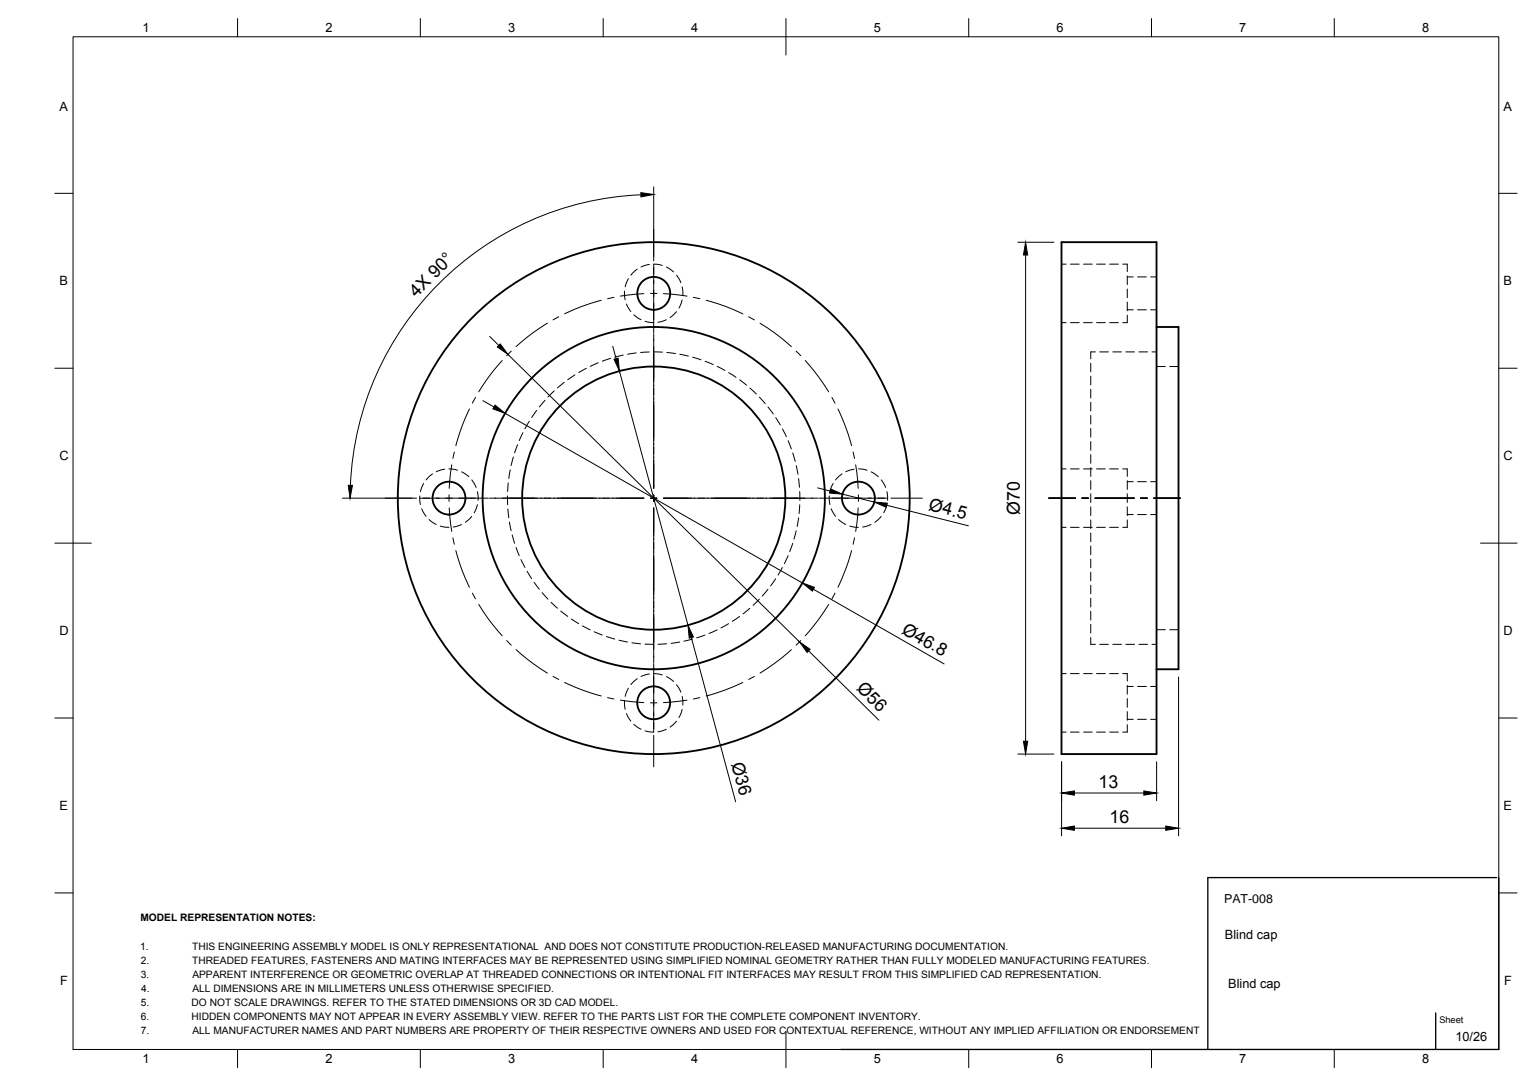
ISO-10303-21;
HEADER;
/* Generated by software containing ST-Developer
 * from STEP Tools, Inc. (www.steptools.com) 
 */

FILE_DESCRIPTION(
/* description */ ('Bearing housing with oil seal and end cap'),
/* implementation_level */ '2;1');

FILE_NAME(
/* name */ 'Blind cap.step',
/* time_stamp */ '2026-10-28T03:23:10-07:00',
/* author */ (''),
/* organization */ (''),
/* preprocessor_version */ 'ST-DEVELOPER v20.2',
/* originating_system */ 'Autodesk Translation Framework v15.17.0.0',
/* authorisation */ '');

FILE_SCHEMA (('AUTOMOTIVE_DESIGN { 1 0 10303 214 3 1 1 }'));
ENDSEC;

DATA;
#10=MECHANICAL_DESIGN_GEOMETRIC_PRESENTATION_REPRESENTATION('',(#264),#7871);
#222=SHAPE_REPRESENTATION_RELATIONSHIP('SRR','None',#7969,#243);
#243=ADVANCED_BREP_SHAPE_REPRESENTATION('',(#293),#7853);
#264=STYLED_ITEM('',(#8146),#293);
#293=MANIFOLD_SOLID_BREP('Body1',#4090);
#359=FACE_BOUND('',#921,.T.);
#360=FACE_BOUND('',#924,.T.);
#361=FACE_BOUND('',#927,.T.);
#362=FACE_BOUND('',#930,.T.);
#363=FACE_BOUND('',#936,.T.);
#364=FACE_BOUND('',#940,.T.);
#365=FACE_BOUND('',#945,.T.);
#366=FACE_BOUND('',#946,.T.);
#367=FACE_BOUND('',#947,.T.);
#368=FACE_BOUND('',#948,.T.);
#369=FACE_BOUND('',#950,.T.);
#370=FACE_BOUND('',#951,.T.);
#371=FACE_BOUND('',#952,.T.);
#372=FACE_BOUND('',#953,.T.);
#373=FACE_BOUND('',#954,.T.);
#450=PLANE('',#4499);
#451=PLANE('',#4504);
#452=PLANE('',#4509);
#453=PLANE('',#4514);
#454=PLANE('',#4524);
#455=PLANE('',#4532);
#456=PLANE('',#4535);
#457=PLANE('',#4539);
#458=PLANE('',#4540);
#624=FACE_OUTER_BOUND('',#919,.T.);
#625=FACE_OUTER_BOUND('',#920,.T.);
#626=FACE_OUTER_BOUND('',#922,.T.);
#627=FACE_OUTER_BOUND('',#923,.T.);
#628=FACE_OUTER_BOUND('',#925,.T.);
#629=FACE_OUTER_BOUND('',#926,.T.);
#630=FACE_OUTER_BOUND('',#928,.T.);
#631=FACE_OUTER_BOUND('',#929,.T.);
#632=FACE_OUTER_BOUND('',#931,.T.);
#633=FACE_OUTER_BOUND('',#932,.T.);
#634=FACE_OUTER_BOUND('',#933,.T.);
#635=FACE_OUTER_BOUND('',#934,.T.);
#636=FACE_OUTER_BOUND('',#935,.T.);
#637=FACE_OUTER_BOUND('',#937,.T.);
#638=FACE_OUTER_BOUND('',#938,.T.);
#639=FACE_OUTER_BOUND('',#939,.T.);
#640=FACE_OUTER_BOUND('',#941,.T.);
#641=FACE_OUTER_BOUND('',#942,.T.);
#642=FACE_OUTER_BOUND('',#943,.T.);
#643=FACE_OUTER_BOUND('',#944,.T.);
#644=FACE_OUTER_BOUND('',#949,.T.);
#919=EDGE_LOOP('',(#3035,#3036,#3037,#3038));
#920=EDGE_LOOP('',(#3039));
#921=EDGE_LOOP('',(#3040));
#922=EDGE_LOOP('',(#3041,#3042,#3043,#3044));
#923=EDGE_LOOP('',(#3045));
#924=EDGE_LOOP('',(#3046));
#925=EDGE_LOOP('',(#3047,#3048,#3049,#3050));
#926=EDGE_LOOP('',(#3051));
#927=EDGE_LOOP('',(#3052));
#928=EDGE_LOOP('',(#3053,#3054,#3055,#3056));
#929=EDGE_LOOP('',(#3057));
#930=EDGE_LOOP('',(#3058));
#931=EDGE_LOOP('',(#3059,#3060,#3061,#3062));
#932=EDGE_LOOP('',(#3063,#3064,#3065,#3066));
#933=EDGE_LOOP('',(#3067,#3068,#3069,#3070));
#934=EDGE_LOOP('',(#3071,#3072,#3073,#3074));
#935=EDGE_LOOP('',(#3075));
#936=EDGE_LOOP('',(#3076));
#937=EDGE_LOOP('',(#3077,#3078,#3079,#3080));
#938=EDGE_LOOP('',(#3081,#3082,#3083,#3084));
#939=EDGE_LOOP('',(#3085));
#940=EDGE_LOOP('',(#3086));
#941=EDGE_LOOP('',(#3087,#3088,#3089,#3090));
#942=EDGE_LOOP('',(#3091));
#943=EDGE_LOOP('',(#3092,#3093,#3094,#3095));
#944=EDGE_LOOP('',(#3096));
#945=EDGE_LOOP('',(#3097));
#946=EDGE_LOOP('',(#3098));
#947=EDGE_LOOP('',(#3099));
#948=EDGE_LOOP('',(#3100));
#949=EDGE_LOOP('',(#3101));
#950=EDGE_LOOP('',(#3102));
#951=EDGE_LOOP('',(#3103));
#952=EDGE_LOOP('',(#3104));
#953=EDGE_LOOP('',(#3105));
#954=EDGE_LOOP('',(#3106));
#1225=LINE('',#6532,#1487);
#1226=LINE('',#6541,#1488);
#1227=LINE('',#6550,#1489);
#1228=LINE('',#6559,#1490);
#1229=LINE('',#6567,#1491);
#1230=LINE('',#6571,#1492);
#1231=LINE('',#6575,#1493);
#1232=LINE('',#6579,#1494);
#1233=LINE('',#6587,#1495);
#1234=LINE('',#6593,#1496);
#1235=LINE('',#6598,#1497);
#1236=LINE('',#6605,#1498);
#1487=VECTOR('',#5258,0.4);
#1488=VECTOR('',#5269,0.4);
#1489=VECTOR('',#5280,0.4);
#1490=VECTOR('',#5291,0.4);
#1491=VECTOR('',#5302,0.225);
#1492=VECTOR('',#5307,0.225);
#1493=VECTOR('',#5312,0.225);
#1494=VECTOR('',#5317,0.225);
#1495=VECTOR('',#5326,1.8);
#1496=VECTOR('',#5333,2.34);
#1497=VECTOR('',#5340,2.);
#1498=VECTOR('',#5349,3.5);
#1739=CIRCLE('',#4497,0.4);
#1740=CIRCLE('',#4498,0.4);
#1741=CIRCLE('',#4500,0.225);
#1742=CIRCLE('',#4502,0.4);
#1743=CIRCLE('',#4503,0.4);
#1744=CIRCLE('',#4505,0.225);
#1745=CIRCLE('',#4507,0.4);
#1746=CIRCLE('',#4508,0.4);
#1747=CIRCLE('',#4510,0.225);
#1748=CIRCLE('',#4512,0.4);
#1749=CIRCLE('',#4513,0.4);
#1750=CIRCLE('',#4515,0.225);
#1751=CIRCLE('',#4517,0.225);
#1752=CIRCLE('',#4519,0.225);
#1753=CIRCLE('',#4521,0.225);
#1754=CIRCLE('',#4523,0.225);
#1755=CIRCLE('',#4525,2.);
#1756=CIRCLE('',#4526,1.8);
#1757=CIRCLE('',#4528,1.8);
#1758=CIRCLE('',#4530,2.34);
#1759=CIRCLE('',#4531,2.34);
#1760=CIRCLE('',#4534,2.);
#1761=CIRCLE('',#4537,3.5);
#1762=CIRCLE('',#4538,3.5);
#1987=VERTEX_POINT('',#6529);
#1988=VERTEX_POINT('',#6531);
#1989=VERTEX_POINT('',#6535);
#1990=VERTEX_POINT('',#6538);
#1991=VERTEX_POINT('',#6540);
#1992=VERTEX_POINT('',#6544);
#1993=VERTEX_POINT('',#6547);
#1994=VERTEX_POINT('',#6549);
#1995=VERTEX_POINT('',#6553);
#1996=VERTEX_POINT('',#6556);
#1997=VERTEX_POINT('',#6558);
#1998=VERTEX_POINT('',#6562);
#1999=VERTEX_POINT('',#6565);
#2000=VERTEX_POINT('',#6569);
#2001=VERTEX_POINT('',#6573);
#2002=VERTEX_POINT('',#6577);
#2003=VERTEX_POINT('',#6581);
#2004=VERTEX_POINT('',#6583);
#2005=VERTEX_POINT('',#6586);
#2006=VERTEX_POINT('',#6590);
#2007=VERTEX_POINT('',#6592);
#2008=VERTEX_POINT('',#6597);
#2009=VERTEX_POINT('',#6602);
#2010=VERTEX_POINT('',#6604);
#2381=EDGE_CURVE('',#1987,#1987,#1739,.T.);
#2382=EDGE_CURVE('',#1987,#1988,#1225,.T.);
#2383=EDGE_CURVE('',#1988,#1988,#1740,.T.);
#2384=EDGE_CURVE('',#1989,#1989,#1741,.T.);
#2385=EDGE_CURVE('',#1990,#1990,#1742,.T.);
#2386=EDGE_CURVE('',#1990,#1991,#1226,.T.);
#2387=EDGE_CURVE('',#1991,#1991,#1743,.T.);
#2388=EDGE_CURVE('',#1992,#1992,#1744,.T.);
#2389=EDGE_CURVE('',#1993,#1993,#1745,.T.);
#2390=EDGE_CURVE('',#1993,#1994,#1227,.T.);
#2391=EDGE_CURVE('',#1994,#1994,#1746,.T.);
#2392=EDGE_CURVE('',#1995,#1995,#1747,.T.);
#2393=EDGE_CURVE('',#1996,#1996,#1748,.T.);
#2394=EDGE_CURVE('',#1996,#1997,#1228,.T.);
#2395=EDGE_CURVE('',#1997,#1997,#1749,.T.);
#2396=EDGE_CURVE('',#1998,#1998,#1750,.T.);
#2397=EDGE_CURVE('',#1999,#1999,#1751,.T.);
#2398=EDGE_CURVE('',#1999,#1989,#1229,.T.);
#2399=EDGE_CURVE('',#2000,#2000,#1752,.T.);
#2400=EDGE_CURVE('',#2000,#1992,#1230,.T.);
#2401=EDGE_CURVE('',#2001,#2001,#1753,.T.);
#2402=EDGE_CURVE('',#2001,#1995,#1231,.T.);
#2403=EDGE_CURVE('',#2002,#2002,#1754,.T.);
#2404=EDGE_CURVE('',#2002,#1998,#1232,.T.);
#2405=EDGE_CURVE('',#2003,#2003,#1755,.T.);
#2406=EDGE_CURVE('',#2004,#2004,#1756,.T.);
#2407=EDGE_CURVE('',#2004,#2005,#1233,.T.);
#2408=EDGE_CURVE('',#2005,#2005,#1757,.T.);
#2409=EDGE_CURVE('',#2006,#2006,#1758,.T.);
#2410=EDGE_CURVE('',#2006,#2007,#1234,.T.);
#2411=EDGE_CURVE('',#2007,#2007,#1759,.T.);
#2412=EDGE_CURVE('',#2003,#2008,#1235,.T.);
#2413=EDGE_CURVE('',#2008,#2008,#1760,.T.);
#2414=EDGE_CURVE('',#2009,#2009,#1761,.T.);
#2415=EDGE_CURVE('',#2009,#2010,#1236,.T.);
#2416=EDGE_CURVE('',#2010,#2010,#1762,.T.);
#3035=ORIENTED_EDGE('',*,*,#2381,.F.);
#3036=ORIENTED_EDGE('',*,*,#2382,.T.);
#3037=ORIENTED_EDGE('',*,*,#2383,.F.);
#3038=ORIENTED_EDGE('',*,*,#2382,.F.);
#3039=ORIENTED_EDGE('',*,*,#2381,.T.);
#3040=ORIENTED_EDGE('',*,*,#2384,.F.);
#3041=ORIENTED_EDGE('',*,*,#2385,.F.);
#3042=ORIENTED_EDGE('',*,*,#2386,.T.);
#3043=ORIENTED_EDGE('',*,*,#2387,.F.);
#3044=ORIENTED_EDGE('',*,*,#2386,.F.);
#3045=ORIENTED_EDGE('',*,*,#2385,.T.);
#3046=ORIENTED_EDGE('',*,*,#2388,.F.);
#3047=ORIENTED_EDGE('',*,*,#2389,.F.);
#3048=ORIENTED_EDGE('',*,*,#2390,.T.);
#3049=ORIENTED_EDGE('',*,*,#2391,.F.);
#3050=ORIENTED_EDGE('',*,*,#2390,.F.);
#3051=ORIENTED_EDGE('',*,*,#2389,.T.);
#3052=ORIENTED_EDGE('',*,*,#2392,.F.);
#3053=ORIENTED_EDGE('',*,*,#2393,.F.);
#3054=ORIENTED_EDGE('',*,*,#2394,.T.);
#3055=ORIENTED_EDGE('',*,*,#2395,.F.);
#3056=ORIENTED_EDGE('',*,*,#2394,.F.);
#3057=ORIENTED_EDGE('',*,*,#2393,.T.);
#3058=ORIENTED_EDGE('',*,*,#2396,.F.);
#3059=ORIENTED_EDGE('',*,*,#2397,.F.);
#3060=ORIENTED_EDGE('',*,*,#2398,.T.);
#3061=ORIENTED_EDGE('',*,*,#2384,.T.);
#3062=ORIENTED_EDGE('',*,*,#2398,.F.);
#3063=ORIENTED_EDGE('',*,*,#2399,.F.);
#3064=ORIENTED_EDGE('',*,*,#2400,.T.);
#3065=ORIENTED_EDGE('',*,*,#2388,.T.);
#3066=ORIENTED_EDGE('',*,*,#2400,.F.);
#3067=ORIENTED_EDGE('',*,*,#2401,.F.);
#3068=ORIENTED_EDGE('',*,*,#2402,.T.);
#3069=ORIENTED_EDGE('',*,*,#2392,.T.);
#3070=ORIENTED_EDGE('',*,*,#2402,.F.);
#3071=ORIENTED_EDGE('',*,*,#2403,.F.);
#3072=ORIENTED_EDGE('',*,*,#2404,.T.);
#3073=ORIENTED_EDGE('',*,*,#2396,.T.);
#3074=ORIENTED_EDGE('',*,*,#2404,.F.);
#3075=ORIENTED_EDGE('',*,*,#2405,.T.);
#3076=ORIENTED_EDGE('',*,*,#2406,.T.);
#3077=ORIENTED_EDGE('',*,*,#2406,.F.);
#3078=ORIENTED_EDGE('',*,*,#2407,.T.);
#3079=ORIENTED_EDGE('',*,*,#2408,.T.);
#3080=ORIENTED_EDGE('',*,*,#2407,.F.);
#3081=ORIENTED_EDGE('',*,*,#2409,.F.);
#3082=ORIENTED_EDGE('',*,*,#2410,.T.);
#3083=ORIENTED_EDGE('',*,*,#2411,.T.);
#3084=ORIENTED_EDGE('',*,*,#2410,.F.);
#3085=ORIENTED_EDGE('',*,*,#2411,.F.);
#3086=ORIENTED_EDGE('',*,*,#2408,.F.);
#3087=ORIENTED_EDGE('',*,*,#2405,.F.);
#3088=ORIENTED_EDGE('',*,*,#2412,.T.);
#3089=ORIENTED_EDGE('',*,*,#2413,.T.);
#3090=ORIENTED_EDGE('',*,*,#2412,.F.);
#3091=ORIENTED_EDGE('',*,*,#2413,.F.);
#3092=ORIENTED_EDGE('',*,*,#2414,.F.);
#3093=ORIENTED_EDGE('',*,*,#2415,.T.);
#3094=ORIENTED_EDGE('',*,*,#2416,.T.);
#3095=ORIENTED_EDGE('',*,*,#2415,.F.);
#3096=ORIENTED_EDGE('',*,*,#2414,.T.);
#3097=ORIENTED_EDGE('',*,*,#2395,.T.);
#3098=ORIENTED_EDGE('',*,*,#2391,.T.);
#3099=ORIENTED_EDGE('',*,*,#2387,.T.);
#3100=ORIENTED_EDGE('',*,*,#2383,.T.);
#3101=ORIENTED_EDGE('',*,*,#2416,.F.);
#3102=ORIENTED_EDGE('',*,*,#2409,.T.);
#3103=ORIENTED_EDGE('',*,*,#2403,.T.);
#3104=ORIENTED_EDGE('',*,*,#2401,.T.);
#3105=ORIENTED_EDGE('',*,*,#2399,.T.);
#3106=ORIENTED_EDGE('',*,*,#2397,.T.);
#3789=CYLINDRICAL_SURFACE('',#4496,0.4);
#3790=CYLINDRICAL_SURFACE('',#4501,0.4);
#3791=CYLINDRICAL_SURFACE('',#4506,0.4);
#3792=CYLINDRICAL_SURFACE('',#4511,0.4);
#3793=CYLINDRICAL_SURFACE('',#4516,0.225);
#3794=CYLINDRICAL_SURFACE('',#4518,0.225);
#3795=CYLINDRICAL_SURFACE('',#4520,0.225);
#3796=CYLINDRICAL_SURFACE('',#4522,0.225);
#3797=CYLINDRICAL_SURFACE('',#4527,1.8);
#3798=CYLINDRICAL_SURFACE('',#4529,2.34);
#3799=CYLINDRICAL_SURFACE('',#4533,2.);
#3800=CYLINDRICAL_SURFACE('',#4536,3.5);
#3906=ADVANCED_FACE('',(#624),#3789,.F.);
#3907=ADVANCED_FACE('',(#625,#359),#450,.T.);
#3908=ADVANCED_FACE('',(#626),#3790,.F.);
#3909=ADVANCED_FACE('',(#627,#360),#451,.T.);
#3910=ADVANCED_FACE('',(#628),#3791,.F.);
#3911=ADVANCED_FACE('',(#629,#361),#452,.T.);
#3912=ADVANCED_FACE('',(#630),#3792,.F.);
#3913=ADVANCED_FACE('',(#631,#362),#453,.T.);
#3914=ADVANCED_FACE('',(#632),#3793,.F.);
#3915=ADVANCED_FACE('',(#633),#3794,.F.);
#3916=ADVANCED_FACE('',(#634),#3795,.F.);
#3917=ADVANCED_FACE('',(#635),#3796,.F.);
#3918=ADVANCED_FACE('',(#636,#363),#454,.T.);
#3919=ADVANCED_FACE('',(#637),#3797,.F.);
#3920=ADVANCED_FACE('',(#638),#3798,.T.);
#3921=ADVANCED_FACE('',(#639,#364),#455,.F.);
#3922=ADVANCED_FACE('',(#640),#3799,.F.);
#3923=ADVANCED_FACE('',(#641),#456,.F.);
#3924=ADVANCED_FACE('',(#642),#3800,.T.);
#3925=ADVANCED_FACE('',(#643,#365,#366,#367,#368),#457,.T.);
#3926=ADVANCED_FACE('',(#644,#369,#370,#371,#372,#373),#458,.F.);
#4090=CLOSED_SHELL('',(#3906,#3907,#3908,#3909,#3910,#3911,#3912,#3913,
#3914,#3915,#3916,#3917,#3918,#3919,#3920,#3921,#3922,#3923,#3924,#3925,
#3926));
#4495=AXIS2_PLACEMENT_3D('',#6527,#5252,#5253);
#4496=AXIS2_PLACEMENT_3D('',#6528,#5254,#5255);
#4497=AXIS2_PLACEMENT_3D('',#6530,#5256,#5257);
#4498=AXIS2_PLACEMENT_3D('',#6533,#5259,#5260);
#4499=AXIS2_PLACEMENT_3D('',#6534,#5261,#5262);
#4500=AXIS2_PLACEMENT_3D('',#6536,#5263,#5264);
#4501=AXIS2_PLACEMENT_3D('',#6537,#5265,#5266);
#4502=AXIS2_PLACEMENT_3D('',#6539,#5267,#5268);
#4503=AXIS2_PLACEMENT_3D('',#6542,#5270,#5271);
#4504=AXIS2_PLACEMENT_3D('',#6543,#5272,#5273);
#4505=AXIS2_PLACEMENT_3D('',#6545,#5274,#5275);
#4506=AXIS2_PLACEMENT_3D('',#6546,#5276,#5277);
#4507=AXIS2_PLACEMENT_3D('',#6548,#5278,#5279);
#4508=AXIS2_PLACEMENT_3D('',#6551,#5281,#5282);
#4509=AXIS2_PLACEMENT_3D('',#6552,#5283,#5284);
#4510=AXIS2_PLACEMENT_3D('',#6554,#5285,#5286);
#4511=AXIS2_PLACEMENT_3D('',#6555,#5287,#5288);
#4512=AXIS2_PLACEMENT_3D('',#6557,#5289,#5290);
#4513=AXIS2_PLACEMENT_3D('',#6560,#5292,#5293);
#4514=AXIS2_PLACEMENT_3D('',#6561,#5294,#5295);
#4515=AXIS2_PLACEMENT_3D('',#6563,#5296,#5297);
#4516=AXIS2_PLACEMENT_3D('',#6564,#5298,#5299);
#4517=AXIS2_PLACEMENT_3D('',#6566,#5300,#5301);
#4518=AXIS2_PLACEMENT_3D('',#6568,#5303,#5304);
#4519=AXIS2_PLACEMENT_3D('',#6570,#5305,#5306);
#4520=AXIS2_PLACEMENT_3D('',#6572,#5308,#5309);
#4521=AXIS2_PLACEMENT_3D('',#6574,#5310,#5311);
#4522=AXIS2_PLACEMENT_3D('',#6576,#5313,#5314);
#4523=AXIS2_PLACEMENT_3D('',#6578,#5315,#5316);
#4524=AXIS2_PLACEMENT_3D('',#6580,#5318,#5319);
#4525=AXIS2_PLACEMENT_3D('',#6582,#5320,#5321);
#4526=AXIS2_PLACEMENT_3D('',#6584,#5322,#5323);
#4527=AXIS2_PLACEMENT_3D('',#6585,#5324,#5325);
#4528=AXIS2_PLACEMENT_3D('',#6588,#5327,#5328);
#4529=AXIS2_PLACEMENT_3D('',#6589,#5329,#5330);
#4530=AXIS2_PLACEMENT_3D('',#6591,#5331,#5332);
#4531=AXIS2_PLACEMENT_3D('',#6594,#5334,#5335);
#4532=AXIS2_PLACEMENT_3D('',#6595,#5336,#5337);
#4533=AXIS2_PLACEMENT_3D('',#6596,#5338,#5339);
#4534=AXIS2_PLACEMENT_3D('',#6599,#5341,#5342);
#4535=AXIS2_PLACEMENT_3D('',#6600,#5343,#5344);
#4536=AXIS2_PLACEMENT_3D('',#6601,#5345,#5346);
#4537=AXIS2_PLACEMENT_3D('',#6603,#5347,#5348);
#4538=AXIS2_PLACEMENT_3D('',#6606,#5350,#5351);
#4539=AXIS2_PLACEMENT_3D('',#6607,#5352,#5353);
#4540=AXIS2_PLACEMENT_3D('',#6608,#5354,#5355);
#5252=DIRECTION('axis',(0.,0.,1.));
#5253=DIRECTION('refdir',(1.,0.,0.));
#5254=DIRECTION('center_axis',(0.,1.,0.));
#5255=DIRECTION('ref_axis',(1.,0.,0.));
#5256=DIRECTION('center_axis',(0.,1.,0.));
#5257=DIRECTION('ref_axis',(1.,0.,0.));
#5258=DIRECTION('',(0.,1.,0.));
#5259=DIRECTION('center_axis',(0.,-1.,0.));
#5260=DIRECTION('ref_axis',(1.,0.,0.));
#5261=DIRECTION('center_axis',(0.,1.,0.));
#5262=DIRECTION('ref_axis',(1.,0.,0.));
#5263=DIRECTION('center_axis',(0.,1.,0.));
#5264=DIRECTION('ref_axis',(1.,0.,0.));
#5265=DIRECTION('center_axis',(0.,1.,0.));
#5266=DIRECTION('ref_axis',(1.,0.,0.));
#5267=DIRECTION('center_axis',(0.,1.,0.));
#5268=DIRECTION('ref_axis',(1.,0.,0.));
#5269=DIRECTION('',(0.,1.,0.));
#5270=DIRECTION('center_axis',(0.,-1.,0.));
#5271=DIRECTION('ref_axis',(1.,0.,0.));
#5272=DIRECTION('center_axis',(0.,1.,0.));
#5273=DIRECTION('ref_axis',(1.,0.,0.));
#5274=DIRECTION('center_axis',(0.,1.,0.));
#5275=DIRECTION('ref_axis',(1.,0.,0.));
#5276=DIRECTION('center_axis',(0.,1.,0.));
#5277=DIRECTION('ref_axis',(1.,0.,0.));
#5278=DIRECTION('center_axis',(0.,1.,0.));
#5279=DIRECTION('ref_axis',(1.,0.,0.));
#5280=DIRECTION('',(0.,1.,0.));
#5281=DIRECTION('center_axis',(0.,-1.,0.));
#5282=DIRECTION('ref_axis',(1.,0.,0.));
#5283=DIRECTION('center_axis',(0.,1.,0.));
#5284=DIRECTION('ref_axis',(1.,0.,0.));
#5285=DIRECTION('center_axis',(0.,1.,0.));
#5286=DIRECTION('ref_axis',(1.,0.,0.));
#5287=DIRECTION('center_axis',(0.,1.,0.));
#5288=DIRECTION('ref_axis',(1.,0.,0.));
#5289=DIRECTION('center_axis',(0.,1.,0.));
#5290=DIRECTION('ref_axis',(1.,0.,0.));
#5291=DIRECTION('',(0.,1.,0.));
#5292=DIRECTION('center_axis',(0.,-1.,0.));
#5293=DIRECTION('ref_axis',(1.,0.,0.));
#5294=DIRECTION('center_axis',(0.,1.,0.));
#5295=DIRECTION('ref_axis',(1.,0.,0.));
#5296=DIRECTION('center_axis',(0.,1.,0.));
#5297=DIRECTION('ref_axis',(1.,0.,0.));
#5298=DIRECTION('center_axis',(0.,1.,0.));
#5299=DIRECTION('ref_axis',(1.,0.,0.));
#5300=DIRECTION('center_axis',(0.,1.,0.));
#5301=DIRECTION('ref_axis',(1.,0.,0.));
#5302=DIRECTION('',(0.,1.,0.));
#5303=DIRECTION('center_axis',(0.,1.,0.));
#5304=DIRECTION('ref_axis',(1.,0.,0.));
#5305=DIRECTION('center_axis',(0.,1.,0.));
#5306=DIRECTION('ref_axis',(1.,0.,0.));
#5307=DIRECTION('',(0.,1.,0.));
#5308=DIRECTION('center_axis',(0.,1.,0.));
#5309=DIRECTION('ref_axis',(1.,0.,0.));
#5310=DIRECTION('center_axis',(0.,1.,0.));
#5311=DIRECTION('ref_axis',(1.,0.,0.));
#5312=DIRECTION('',(0.,1.,0.));
#5313=DIRECTION('center_axis',(0.,1.,0.));
#5314=DIRECTION('ref_axis',(1.,0.,0.));
#5315=DIRECTION('center_axis',(0.,1.,0.));
#5316=DIRECTION('ref_axis',(1.,0.,0.));
#5317=DIRECTION('',(0.,1.,0.));
#5318=DIRECTION('center_axis',(0.,1.,0.));
#5319=DIRECTION('ref_axis',(1.,0.,0.));
#5320=DIRECTION('center_axis',(0.,1.,0.));
#5321=DIRECTION('ref_axis',(1.,0.,0.));
#5322=DIRECTION('center_axis',(0.,-1.,0.));
#5323=DIRECTION('ref_axis',(1.,0.,0.));
#5324=DIRECTION('center_axis',(0.,1.,0.));
#5325=DIRECTION('ref_axis',(1.,0.,0.));
#5326=DIRECTION('',(0.,-1.,0.));
#5327=DIRECTION('center_axis',(0.,-1.,0.));
#5328=DIRECTION('ref_axis',(1.,0.,0.));
#5329=DIRECTION('center_axis',(0.,1.,0.));
#5330=DIRECTION('ref_axis',(1.,0.,0.));
#5331=DIRECTION('center_axis',(0.,1.,0.));
#5332=DIRECTION('ref_axis',(1.,0.,0.));
#5333=DIRECTION('',(0.,-1.,0.));
#5334=DIRECTION('center_axis',(0.,1.,0.));
#5335=DIRECTION('ref_axis',(1.,0.,0.));
#5336=DIRECTION('center_axis',(0.,1.,0.));
#5337=DIRECTION('ref_axis',(1.,0.,0.));
#5338=DIRECTION('center_axis',(0.,1.,0.));
#5339=DIRECTION('ref_axis',(1.,0.,0.));
#5340=DIRECTION('',(0.,1.,0.));
#5341=DIRECTION('center_axis',(0.,1.,0.));
#5342=DIRECTION('ref_axis',(1.,0.,0.));
#5343=DIRECTION('center_axis',(0.,1.,0.));
#5344=DIRECTION('ref_axis',(1.,0.,0.));
#5345=DIRECTION('center_axis',(0.,1.,0.));
#5346=DIRECTION('ref_axis',(1.,0.,0.));
#5347=DIRECTION('center_axis',(0.,1.,0.));
#5348=DIRECTION('ref_axis',(1.,0.,0.));
#5349=DIRECTION('',(0.,-1.,0.));
#5350=DIRECTION('center_axis',(0.,1.,0.));
#5351=DIRECTION('ref_axis',(1.,0.,0.));
#5352=DIRECTION('center_axis',(0.,1.,0.));
#5353=DIRECTION('ref_axis',(1.,0.,0.));
#5354=DIRECTION('center_axis',(0.,1.,0.));
#5355=DIRECTION('ref_axis',(1.,0.,0.));
#6527=CARTESIAN_POINT('',(0.,0.,0.));
#6528=CARTESIAN_POINT('Origin',(-2.8,6.4,4.5));
#6529=CARTESIAN_POINT('',(-3.2,6.4,4.5));
#6530=CARTESIAN_POINT('Origin',(-2.8,6.4,4.5));
#6531=CARTESIAN_POINT('',(-3.2,7.3,4.5));
#6532=CARTESIAN_POINT('',(-3.2,6.4,4.5));
#6533=CARTESIAN_POINT('Origin',(-2.8,7.3,4.5));
#6534=CARTESIAN_POINT('Origin',(-2.8,6.4,4.5));
#6535=CARTESIAN_POINT('',(-3.025,6.4,4.5));
#6536=CARTESIAN_POINT('Origin',(-2.8,6.4,4.5));
#6537=CARTESIAN_POINT('Origin',(1.71450551880629E-16,6.4,7.3));
#6538=CARTESIAN_POINT('',(-0.4,6.4,7.3));
#6539=CARTESIAN_POINT('Origin',(1.71450551880629E-16,6.4,7.3));
#6540=CARTESIAN_POINT('',(-0.4,7.3,7.3));
#6541=CARTESIAN_POINT('',(-0.4,6.4,7.3));
#6542=CARTESIAN_POINT('Origin',(1.71450551880629E-16,7.3,7.3));
#6543=CARTESIAN_POINT('Origin',(1.66533453693773E-16,6.4,7.3));
#6544=CARTESIAN_POINT('',(-0.225,6.4,7.3));
#6545=CARTESIAN_POINT('Origin',(1.71450551880629E-16,6.4,7.3));
#6546=CARTESIAN_POINT('Origin',(2.8,6.4,4.5));
#6547=CARTESIAN_POINT('',(2.4,6.4,4.5));
#6548=CARTESIAN_POINT('Origin',(2.8,6.4,4.5));
#6549=CARTESIAN_POINT('',(2.4,7.3,4.5));
#6550=CARTESIAN_POINT('',(2.4,6.4,4.5));
#6551=CARTESIAN_POINT('Origin',(2.8,7.3,4.5));
#6552=CARTESIAN_POINT('Origin',(2.8,6.4,4.5));
#6553=CARTESIAN_POINT('',(2.575,6.4,4.5));
#6554=CARTESIAN_POINT('Origin',(2.8,6.4,4.5));
#6555=CARTESIAN_POINT('Origin',(-5.14351655641888E-16,6.4,1.7));
#6556=CARTESIAN_POINT('',(-0.400000000000001,6.4,1.7));
#6557=CARTESIAN_POINT('Origin',(-5.14351655641888E-16,6.4,1.7));
#6558=CARTESIAN_POINT('',(-0.400000000000001,7.3,1.7));
#6559=CARTESIAN_POINT('',(-0.400000000000001,6.4,1.7));
#6560=CARTESIAN_POINT('Origin',(-5.14351655641888E-16,7.3,1.7));
#6561=CARTESIAN_POINT('Origin',(-4.9960036108132E-16,6.4,1.7));
#6562=CARTESIAN_POINT('',(-0.225000000000001,6.4,1.7));
#6563=CARTESIAN_POINT('Origin',(-5.14351655641888E-16,6.4,1.7));
#6564=CARTESIAN_POINT('Origin',(-2.8,5.9,4.5));
#6565=CARTESIAN_POINT('',(-3.025,6.,4.5));
#6566=CARTESIAN_POINT('Origin',(-2.8,6.,4.5));
#6567=CARTESIAN_POINT('',(-3.025,5.9,4.5));
#6568=CARTESIAN_POINT('Origin',(1.71450551880629E-16,5.9,7.3));
#6569=CARTESIAN_POINT('',(-0.225,6.,7.3));
#6570=CARTESIAN_POINT('Origin',(1.71450551880629E-16,6.,7.3));
#6571=CARTESIAN_POINT('',(-0.225,5.9,7.3));
#6572=CARTESIAN_POINT('Origin',(2.8,5.9,4.5));
#6573=CARTESIAN_POINT('',(2.575,6.,4.5));
#6574=CARTESIAN_POINT('Origin',(2.8,6.,4.5));
#6575=CARTESIAN_POINT('',(2.575,5.9,4.5));
#6576=CARTESIAN_POINT('Origin',(-5.14351655641888E-16,5.9,1.7));
#6577=CARTESIAN_POINT('',(-0.225000000000001,6.,1.7));
#6578=CARTESIAN_POINT('Origin',(-5.14351655641888E-16,6.,1.7));
#6579=CARTESIAN_POINT('',(-0.225000000000001,5.9,1.7));
#6580=CARTESIAN_POINT('Origin',(0.,6.,4.5));
#6581=CARTESIAN_POINT('',(-2.,6.,4.5));
#6582=CARTESIAN_POINT('Origin',(0.,6.,4.5));
#6583=CARTESIAN_POINT('',(-1.8,6.,4.5));
#6584=CARTESIAN_POINT('Origin',(0.,6.,4.5));
#6585=CARTESIAN_POINT('Origin',(0.,5.7,4.5));
#6586=CARTESIAN_POINT('',(-1.8,5.7,4.5));
#6587=CARTESIAN_POINT('',(-1.8,5.7,4.5));
#6588=CARTESIAN_POINT('Origin',(0.,5.7,4.5));
#6589=CARTESIAN_POINT('Origin',(0.,5.7,4.5));
#6590=CARTESIAN_POINT('',(-2.34,6.,4.5));
#6591=CARTESIAN_POINT('Origin',(0.,6.,4.5));
#6592=CARTESIAN_POINT('',(-2.34,5.7,4.5));
#6593=CARTESIAN_POINT('',(-2.34,5.7,4.5));
#6594=CARTESIAN_POINT('Origin',(0.,5.7,4.5));
#6595=CARTESIAN_POINT('Origin',(0.,5.7,4.5));
#6596=CARTESIAN_POINT('Origin',(0.,5.9,4.5));
#6597=CARTESIAN_POINT('',(-2.,6.9,4.5));
#6598=CARTESIAN_POINT('',(-2.,5.9,4.5));
#6599=CARTESIAN_POINT('Origin',(0.,6.9,4.5));
#6600=CARTESIAN_POINT('Origin',(0.,6.9,4.5));
#6601=CARTESIAN_POINT('Origin',(0.,6.,4.5));
#6602=CARTESIAN_POINT('',(-3.5,7.3,4.5));
#6603=CARTESIAN_POINT('Origin',(0.,7.3,4.5));
#6604=CARTESIAN_POINT('',(-3.5,6.,4.5));
#6605=CARTESIAN_POINT('',(-3.5,6.,4.5));
#6606=CARTESIAN_POINT('Origin',(0.,6.,4.5));
#6607=CARTESIAN_POINT('Origin',(0.,7.3,4.5));
#6608=CARTESIAN_POINT('Origin',(0.,6.,4.5));
#7827=UNCERTAINTY_MEASURE_WITH_UNIT(LENGTH_MEASURE(0.001),#7872,
'DISTANCE_ACCURACY_VALUE',
'Maximum model space distance between geometric entities at asserted c
onnectivities');
#7845=UNCERTAINTY_MEASURE_WITH_UNIT(LENGTH_MEASURE(0.001),#7872,
'DISTANCE_ACCURACY_VALUE',
'Maximum model space distance between geometric entities at asserted c
onnectivities');
#7853=(
GEOMETRIC_REPRESENTATION_CONTEXT(3)
GLOBAL_UNCERTAINTY_ASSIGNED_CONTEXT((#7827))
GLOBAL_UNIT_ASSIGNED_CONTEXT((#7872,#7874,#7875))
REPRESENTATION_CONTEXT('','3D')
);
#7871=(
GEOMETRIC_REPRESENTATION_CONTEXT(3)
GLOBAL_UNCERTAINTY_ASSIGNED_CONTEXT((#7845))
GLOBAL_UNIT_ASSIGNED_CONTEXT((#7872,#7874,#7875))
REPRESENTATION_CONTEXT('','3D')
);
#7872=(
LENGTH_UNIT()
NAMED_UNIT(*)
SI_UNIT(.CENTI.,.METRE.)
);
#7874=(
NAMED_UNIT(*)
PLANE_ANGLE_UNIT()
SI_UNIT($,.RADIAN.)
);
#7875=(
NAMED_UNIT(*)
SI_UNIT($,.STERADIAN.)
SOLID_ANGLE_UNIT()
);
#7883=SHAPE_DEFINITION_REPRESENTATION(#7908,#7969);
#7908=PRODUCT_DEFINITION_SHAPE('',$,#7995);
#7969=SHAPE_REPRESENTATION('',(#4495),#7853);
#7987=PRODUCT_DEFINITION_CONTEXT('part definition',#8064,'design');
#7995=PRODUCT_DEFINITION('Blind cap','Blind cap',#8020,#7987);
#8020=PRODUCT_DEFINITION_FORMATION('',$,#8073);
#8064=APPLICATION_CONTEXT(
'Core Data for Automotive Mechanical Design Process');
#8065=PRODUCT_CONTEXT('part definition',#8064,'mechanical');
#8073=PRODUCT('Blind cap','Blind cap','Blind cap',(#8065));
#8140=COLOUR_RGB('Sky Blue',0.24,0.69,0.87);
#8141=FILL_AREA_STYLE_COLOUR('',#8140);
#8142=FILL_AREA_STYLE('',(#8141));
#8143=SURFACE_STYLE_FILL_AREA(#8142);
#8144=SURFACE_SIDE_STYLE('',(#8143));
#8145=SURFACE_STYLE_USAGE(.BOTH.,#8144);
#8146=PRESENTATION_STYLE_ASSIGNMENT((#8145));
ENDSEC;
END-ISO-10303-21;
